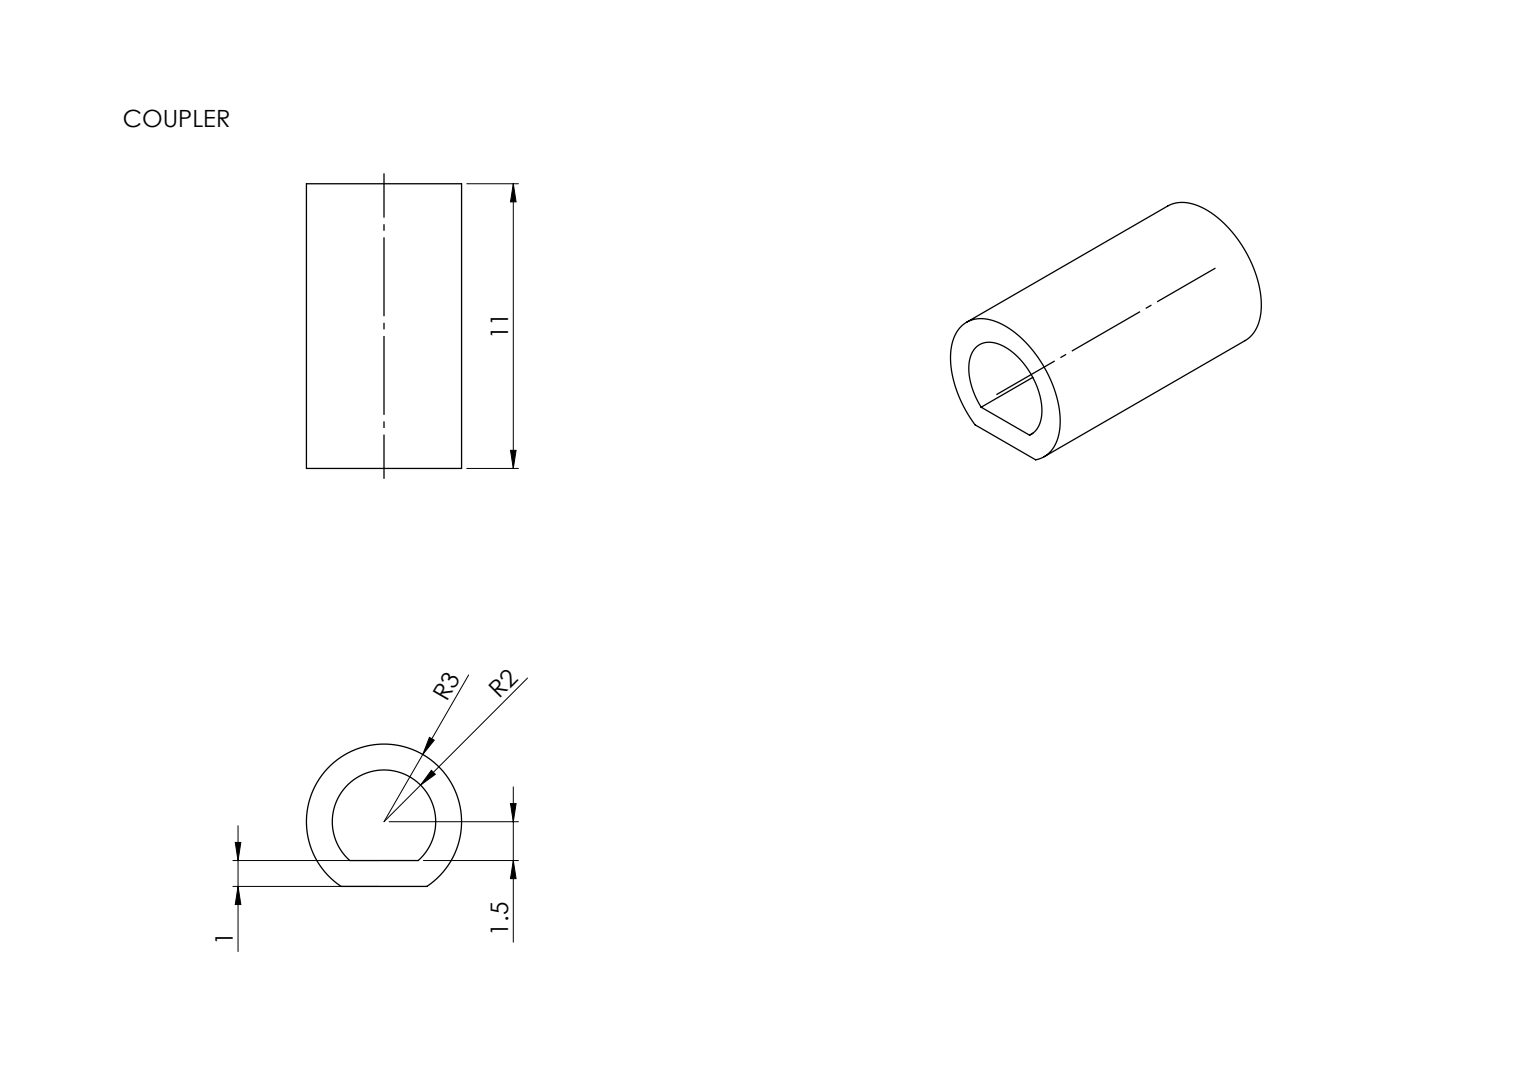
ISO-10303-21;
HEADER;
FILE_DESCRIPTION (('STEP AP214'),
    '1' );
FILE_NAME ('coupler.step',
    '2026-10-02T09:26:43',
    ( '' ),
    ( '' ),
    'SwSTEP 2.0',
    'SolidWorks 2026',
    '' );
FILE_SCHEMA (( 'AUTOMOTIVE_DESIGN' ));
ENDSEC;

DATA;
#121=CARTESIAN_POINT ( 'NONE',  ( -3.000000000000000000, 3.673940397442059868E-16, -5.000000000000004441 ) ) ;
#140=FACE_OUTER_BOUND ( 'NONE', #29426, .T. ) ;
#510=CARTESIAN_POINT ( 'NONE',  ( 0.000000000000000000, 0.000000000000000000, 6.000000000000005329 ) ) ;
#797=DIRECTION ( 'NONE',  ( 0.000000000000000000, -1.000000000000000000, 0.000000000000000000 ) ) ;
#830=EDGE_CURVE ( 'NONE', #63242, #121356, #72655, .T. ) ;
#3162=DIRECTION ( 'NONE',  ( 1.000000000000000000, 0.000000000000000000, 0.000000000000000000 ) ) ;
#3336=EDGE_CURVE ( 'NONE', #106026, #55502, #20118, .T. ) ;
#3524=CARTESIAN_POINT ( 'NONE',  ( -3.000000000000000000, 3.673940397442059868E-16, 6.000000000000005329 ) ) ;
#3829=VECTOR ( 'NONE', #31652, 1000.000000000000000 ) ;
#3916=SHAPE_REPRESENTATION_RELATIONSHIP ( 'NONE' , 'NONE' ,  #71195, #50879 ) ;
#4519=PRODUCT_DEFINITION_FORMATION_WITH_SPECIFIED_SOURCE ( 'ANY', '', #111975, .NOT_KNOWN. ) ;
#5236=PRODUCT_DEFINITION ( 'UNKNOWN', '', #4519, #49332 ) ;
#5531=AXIS2_PLACEMENT_3D ( 'NONE', #87883, #67606, #9346 ) ;
#5667=AXIS2_PLACEMENT_3D ( 'NONE', #39891, #58867, #98137 ) ;
#5700=CARTESIAN_POINT ( 'NONE',  ( -1.322875655532295136, -1.500000000000000222, 6.000000000000005329 ) ) ;
#5791=EDGE_LOOP ( 'NONE', ( #54468, #103310, #17198, #105823 ) ) ;
#6026=AXIS2_PLACEMENT_3D ( 'NONE', #62055, #31948, #71212 ) ;
#6057=FILL_AREA_STYLE_COLOUR ( '', #69146 ) ;
#6824=DIRECTION ( 'NONE',  ( 0.000000000000000000, 0.000000000000000000, 1.000000000000000000 ) ) ;
#6973=EDGE_CURVE ( 'NONE', #15557, #33416, #50411, .T. ) ;
#7096=EDGE_CURVE ( 'NONE', #113294, #58747, #13842, .T. ) ;
#7288=ORIENTED_EDGE ( 'NONE', *, *, #129076, .T. ) ;
#7517=CIRCLE ( 'NONE', #99487, 2.000000000000000000 ) ;
#8386=EDGE_LOOP ( 'NONE', ( #21515, #31620, #80877, #68622 ) ) ;
#8391=ADVANCED_FACE ( 'NONE', ( #66505 ), #113691, .T. ) ;
#8628=PRESENTATION_STYLE_ASSIGNMENT (( #46012 ) ) ;
#9105=VERTEX_POINT ( 'NONE', #120623 ) ;
#9346=DIRECTION ( 'NONE',  ( 1.000000000000000000, 0.000000000000000000, 0.000000000000000000 ) ) ;
#10644=CARTESIAN_POINT ( 'NONE',  ( 0.000000000000000000, 0.000000000000000000, 0.000000000000000000 ) ) ;
#10879=ORIENTED_EDGE ( 'NONE', *, *, #26098, .F. ) ;
#11137=DIRECTION ( 'NONE',  ( 0.000000000000000000, 0.000000000000000000, -1.000000000000000000 ) ) ;
#11803=VECTOR ( 'NONE', #66278, 1000.000000000000000 ) ;
#12273=CARTESIAN_POINT ( 'NONE',  ( 0.000000000000000000, 0.000000000000000000, 6.000000000000005329 ) ) ;
#12515=CARTESIAN_POINT ( 'NONE',  ( 0.000000000000000000, 0.000000000000000000, 6.000000000000005329 ) ) ;
#12752=VERTEX_POINT ( 'NONE', #40215 ) ;
#13727=PRESENTATION_STYLE_ASSIGNMENT (( #105348 ) ) ;
#13796=EDGE_CURVE ( 'NONE', #113294, #14153, #20257, .T. ) ;
#13842=CIRCLE ( 'NONE', #95430, 3.000000000000000000 ) ;
#14153=VERTEX_POINT ( 'NONE', #3524 ) ;
#14367=FILL_AREA_STYLE_COLOUR ( '', #49923 ) ;
#15427=DIRECTION ( 'NONE',  ( 0.000000000000000000, 0.000000000000000000, 1.000000000000000000 ) ) ;
#15480=ORIENTED_EDGE ( 'NONE', *, *, #26098, .T. ) ;
#15494=CARTESIAN_POINT ( 'NONE',  ( 0.000000000000000000, 0.000000000000000000, -5.000000000000004441 ) ) ;
#15557=VERTEX_POINT ( 'NONE', #69207 ) ;
#15625=EDGE_LOOP ( 'NONE', ( #57211, #65939, #124671, #93586 ) ) ;
#15810=VECTOR ( 'NONE', #20956, 1000.000000000000000 ) ;
#16030=ADVANCED_FACE ( 'NONE', ( #40541 ), #18290, .F. ) ;
#16169=AXIS2_PLACEMENT_3D ( 'NONE', #75260, #26171, #96181 ) ;
#16469=ORIENTED_EDGE ( 'NONE', *, *, #30069, .F. ) ;
#16559=FACE_BOUND ( 'NONE', #42887, .T. ) ;
#16568=EDGE_CURVE ( 'NONE', #33416, #14153, #125380, .T. ) ;
#16696=EDGE_LOOP ( 'NONE', ( #90752, #119802, #97487, #87277 ) ) ;
#16932=VERTEX_POINT ( 'NONE', #51031 ) ;
#17198=ORIENTED_EDGE ( 'NONE', *, *, #76465, .F. ) ;
#18290=CYLINDRICAL_SURFACE ( 'NONE', #5667, 2.000000000000000000 ) ;
#18737=ORIENTED_EDGE ( 'NONE', *, *, #42194, .F. ) ;
#18894=ORIENTED_EDGE ( 'NONE', *, *, #67726, .F. ) ;
#19635=FACE_OUTER_BOUND ( 'NONE', #8386, .T. ) ;
#20118=CIRCLE ( 'NONE', #16169, 2.000000000000000000 ) ;
#20257=LINE ( 'NONE', #113632, #62540 ) ;
#20956=DIRECTION ( 'NONE',  ( 0.000000000000000000, 0.000000000000000000, 1.000000000000000000 ) ) ;
#21257=EDGE_CURVE ( 'NONE', #14153, #63242, #113529, .T. ) ;
#21274=VERTEX_POINT ( 'NONE', #79105 ) ;
#21515=ORIENTED_EDGE ( 'NONE', *, *, #13796, .F. ) ;
#21809=CARTESIAN_POINT ( 'NONE',  ( 0.000000000000000000, 0.000000000000000000, 6.000000000000005329 ) ) ;
#22053=AXIS2_PLACEMENT_3D ( 'NONE', #65765, #6824, #24563 ) ;
#22460=DIRECTION ( 'NONE',  ( 0.000000000000000000, 0.000000000000000000, 1.000000000000000000 ) ) ;
#23295=LINE ( 'NONE', #110392, #33797 ) ;
#23792=CARTESIAN_POINT ( 'NONE',  ( 1.322875655532295136, -1.500000000000000222, -5.000000000000004441 ) ) ;
#24563=DIRECTION ( 'NONE',  ( 1.000000000000000000, 0.000000000000000000, 0.000000000000000000 ) ) ;
#24625=APPLICATION_CONTEXT ( 'automotive_design' ) ;
#25196=VECTOR ( 'NONE', #34094, 1000.000000000000000 ) ;
#25601=CIRCLE ( 'NONE', #63187, 2.000000000000000000 ) ;
#26098=EDGE_CURVE ( 'NONE', #15557, #113294, #55419, .T. ) ;
#26171=DIRECTION ( 'NONE',  ( 0.000000000000000000, 0.000000000000000000, 1.000000000000000000 ) ) ;
#26869=DIRECTION ( 'NONE',  ( 1.000000000000000000, 0.000000000000000000, 0.000000000000000000 ) ) ;
#26920=ORIENTED_EDGE ( 'NONE', *, *, #77354, .F. ) ;
#27012=SURFACE_SIDE_STYLE ('',( #58415 ) ) ;
#28342=DIRECTION ( 'NONE',  ( 0.000000000000000000, 0.000000000000000000, -1.000000000000000000 ) ) ;
#28589=EDGE_CURVE ( 'NONE', #16932, #21274, #25601, .T. ) ;
#28709=DIRECTION ( 'NONE',  ( 0.000000000000000000, 0.000000000000000000, 1.000000000000000000 ) ) ;
#28826=AXIS2_PLACEMENT_3D ( 'NONE', #15494, #115628, #103896 ) ;
#28851=AXIS2_PLACEMENT_3D ( 'NONE', #35147, #44955, #56039 ) ;
#28949=ORIENTED_EDGE ( 'NONE', *, *, #117304, .F. ) ;
#28951=LINE ( 'NONE', #86559, #11803 ) ;
#29426=EDGE_LOOP ( 'NONE', ( #127737, #47956, #18737, #67731 ) ) ;
#29661=ORIENTED_EDGE ( 'NONE', *, *, #3336, .T. ) ;
#30069=EDGE_CURVE ( 'NONE', #61997, #15557, #65779, .T. ) ;
#31620=ORIENTED_EDGE ( 'NONE', *, *, #7096, .T. ) ;
#31652=DIRECTION ( 'NONE',  ( 1.000000000000000000, 0.000000000000000000, 0.000000000000000000 ) ) ;
#31948=DIRECTION ( 'NONE',  ( 0.000000000000000000, 0.000000000000000000, 1.000000000000000000 ) ) ;
#32102=DIRECTION ( 'NONE',  ( 0.000000000000000000, -1.000000000000000000, 0.000000000000000000 ) ) ;
#33280=DIRECTION ( 'NONE',  ( 0.000000000000000000, 0.000000000000000000, 1.000000000000000000 ) ) ;
#33402=( NAMED_UNIT ( * ) PLANE_ANGLE_UNIT ( ) SI_UNIT ( $, .RADIAN. ) );
#33416=VERTEX_POINT ( 'NONE', #37331 ) ;
#33552=DIRECTION ( 'NONE',  ( 0.000000000000000000, 0.000000000000000000, 1.000000000000000000 ) ) ;
#33797=VECTOR ( 'NONE', #92044, 1000.000000000000000 ) ;
#33972=EDGE_LOOP ( 'NONE', ( #15480, #69240, #68935, #118863 ) ) ;
#34094=DIRECTION ( 'NONE',  ( 0.000000000000000000, 0.000000000000000000, 1.000000000000000000 ) ) ;
#34695=CARTESIAN_POINT ( 'NONE',  ( -1.658312395177699017, -2.500000000000000444, 6.000000000000005329 ) ) ;
#34746=ADVANCED_FACE ( 'NONE', ( #19635 ), #79830, .T. ) ;
#35092=DIRECTION ( 'NONE',  ( 1.000000000000000000, 0.000000000000000000, 0.000000000000000000 ) ) ;
#35147=CARTESIAN_POINT ( 'NONE',  ( 0.000000000000000000, 0.000000000000000000, -5.000000000000004441 ) ) ;
#35414=LINE ( 'NONE', #125072, #105460 ) ;
#37331=CARTESIAN_POINT ( 'NONE',  ( 3.000000000000000000, 0.000000000000000000, 6.000000000000005329 ) ) ;
#37649=PRODUCT_DEFINITION_SHAPE ( 'NONE', 'NONE',  #5236 ) ;
#37995=APPLICATION_CONTEXT ( 'automotive_design' ) ;
#38839=CYLINDRICAL_SURFACE ( 'NONE', #5531, 2.000000000000000000 ) ;
#39891=CARTESIAN_POINT ( 'NONE',  ( 0.000000000000000000, 0.000000000000000000, -5.000000000000004441 ) ) ;
#40215=CARTESIAN_POINT ( 'NONE',  ( 1.322875655532295136, -1.500000000000000222, 6.000000000000005329 ) ) ;
#40409=CARTESIAN_POINT ( 'NONE',  ( -2.000000000000000000, 2.449293598294706414E-16, 6.000000000000005329 ) ) ;
#40541=FACE_OUTER_BOUND ( 'NONE', #15625, .T. ) ;
#40667=ORIENTED_EDGE ( 'NONE', *, *, #122642, .T. ) ;
#41296=AXIS2_PLACEMENT_3D ( 'NONE', #21809, #22460, #51910 ) ;
#42194=EDGE_CURVE ( 'NONE', #58747, #63242, #35414, .T. ) ;
#42640=EDGE_CURVE ( 'NONE', #21274, #106026, #65167, .T. ) ;
#42657=DIRECTION ( 'NONE',  ( 0.000000000000000000, 0.000000000000000000, 1.000000000000000000 ) ) ;
#42887=EDGE_LOOP ( 'NONE', ( #18894, #74442, #28949, #116817 ) ) ;
#43089=ADVANCED_FACE ( 'NONE', ( #65011, #16559 ), #86602, .T. ) ;
#43736=LINE ( 'NONE', #5700, #55418 ) ;
#43866=SURFACE_STYLE_FILL_AREA ( #84413 ) ;
#44955=DIRECTION ( 'NONE',  ( 0.000000000000000000, 0.000000000000000000, 1.000000000000000000 ) ) ;
#44985=CYLINDRICAL_SURFACE ( 'NONE', #28826, 3.000000000000000000 ) ;
#45200=ORIENTED_EDGE ( 'NONE', *, *, #86954, .F. ) ;
#45468=AXIS2_PLACEMENT_3D ( 'NONE', #12273, #60750, #103252 ) ;
#45745=EDGE_LOOP ( 'NONE', ( #40667, #7288, #88586, #87697 ) ) ;
#45875=CARTESIAN_POINT ( 'NONE',  ( 0.000000000000000000, 0.000000000000000000, -5.000000000000004441 ) ) ;
#46012=SURFACE_STYLE_USAGE ( .BOTH. , #27012 ) ;
#46496=CYLINDRICAL_SURFACE ( 'NONE', #128338, 2.000000000000000000 ) ;
#46647=( NAMED_UNIT ( * ) PLANE_ANGLE_UNIT ( ) SI_UNIT ( $, .RADIAN. ) );
#46771=VECTOR ( 'NONE', #35092, 1000.000000000000000 ) ;
#47956=ORIENTED_EDGE ( 'NONE', *, *, #830, .F. ) ;
#48256=CARTESIAN_POINT ( 'NONE',  ( -1.322875655532295136, -1.500000000000000222, -5.000000000000004441 ) ) ;
#48698=ADVANCED_FACE ( 'NONE', ( #140 ), #69535, .T. ) ;
#48839=AXIS2_PLACEMENT_3D ( 'NONE', #102687, #62788, #73241 ) ;
#49332=PRODUCT_DEFINITION_CONTEXT ( 'detailed design', #24625, 'design' ) ;
#49923=COLOUR_RGB ( '', 0.31764706, 0.68627451, 0.89019608) ;
#50411=LINE ( 'NONE', #110621, #15810 ) ;
#50879=ADVANCED_BREP_SHAPE_REPRESENTATION ( '', ( #102059, #108296 ), #66615 ) ;
#51031=CARTESIAN_POINT ( 'NONE',  ( 2.000000000000000000, 0.000000000000000000, -5.000000000000004441 ) ) ;
#51805=LINE ( 'NONE', #113280, #25196 ) ;
#51910=DIRECTION ( 'NONE',  ( 1.000000000000000000, 0.000000000000000000, 0.000000000000000000 ) ) ;
#54468=ORIENTED_EDGE ( 'NONE', *, *, #77354, .T. ) ;
#54686=CARTESIAN_POINT ( 'NONE',  ( -1.322875655532295136, -2.500000000000000444, -5.000000000000004441 ) ) ;
#55093=DIRECTION ( 'NONE',  ( 1.000000000000000000, 0.000000000000000000, 0.000000000000000000 ) ) ;
#55418=VECTOR ( 'NONE', #73174, 1000.000000000000000 ) ;
#55419=CIRCLE ( 'NONE', #93078, 3.000000000000000000 ) ;
#55502=VERTEX_POINT ( 'NONE', #76988 ) ;
#55575=DIRECTION ( 'NONE',  ( 1.000000000000000000, 0.000000000000000000, 0.000000000000000000 ) ) ;
#55759=ORIENTED_EDGE ( 'NONE', *, *, #7096, .F. ) ;
#56004=CARTESIAN_POINT ( 'NONE',  ( -2.000000000000000000, 2.449293598294706414E-16, -5.000000000000004441 ) ) ;
#56039=DIRECTION ( 'NONE',  ( 1.000000000000000000, 0.000000000000000000, 0.000000000000000000 ) ) ;
#56171=ADVANCED_FACE ( 'NONE', ( #61557 ), #72662, .F. ) ;
#56497=EDGE_CURVE ( 'NONE', #121356, #33416, #57977, .T. ) ;
#56639=ADVANCED_FACE ( 'NONE', ( #75078 ), #44985, .T. ) ;
#56862=DIRECTION ( 'NONE',  ( 1.000000000000000000, 0.000000000000000000, 0.000000000000000000 ) ) ;
#56949=FACE_OUTER_BOUND ( 'NONE', #128515, .T. ) ;
#57211=ORIENTED_EDGE ( 'NONE', *, *, #112117, .F. ) ;
#57977=CIRCLE ( 'NONE', #45468, 3.000000000000000000 ) ;
#58415=SURFACE_STYLE_FILL_AREA ( #127777 ) ;
#58747=VERTEX_POINT ( 'NONE', #58949 ) ;
#58867=DIRECTION ( 'NONE',  ( 0.000000000000000000, 0.000000000000000000, 1.000000000000000000 ) ) ;
#58949=CARTESIAN_POINT ( 'NONE',  ( -1.658312395177699017, -2.500000000000000444, -5.000000000000004441 ) ) ;
#58992=EDGE_CURVE ( 'NONE', #58747, #61997, #83540, .T. ) ;
#59479=DIRECTION ( 'NONE',  ( 1.000000000000000000, 0.000000000000000000, 0.000000000000000000 ) ) ;
#60394=CARTESIAN_POINT ( 'NONE',  ( -1.322875655532295136, -2.500000000000000444, -5.000000000000004441 ) ) ;
#60750=DIRECTION ( 'NONE',  ( 0.000000000000000000, 0.000000000000000000, 1.000000000000000000 ) ) ;
#60816=ADVANCED_FACE ( 'NONE', ( #128505 ), #38839, .F. ) ;
#61198=DIRECTION ( 'NONE',  ( 0.000000000000000000, 0.000000000000000000, 1.000000000000000000 ) ) ;
#61557=FACE_OUTER_BOUND ( 'NONE', #5791, .T. ) ;
#61997=VERTEX_POINT ( 'NONE', #122067 ) ;
#62055=CARTESIAN_POINT ( 'NONE',  ( 0.000000000000000000, 0.000000000000000000, -5.000000000000004441 ) ) ;
#62540=VECTOR ( 'NONE', #99475, 1000.000000000000000 ) ;
#62788=DIRECTION ( 'NONE',  ( 0.000000000000000000, 0.000000000000000000, 1.000000000000000000 ) ) ;
#63187=AXIS2_PLACEMENT_3D ( 'NONE', #126277, #124346, #56862 ) ;
#63242=VERTEX_POINT ( 'NONE', #34695 ) ;
#63328=FACE_BOUND ( 'NONE', #45745, .T. ) ;
#63794=VECTOR ( 'NONE', #15427, 1000.000000000000000 ) ;
#63815=CIRCLE ( 'NONE', #22053, 2.000000000000000000 ) ;
#64736=VECTOR ( 'NONE', #33552, 1000.000000000000000 ) ;
#64852=DIRECTION ( 'NONE',  ( 0.000000000000000000, 0.000000000000000000, 1.000000000000000000 ) ) ;
#64894=CARTESIAN_POINT ( 'NONE',  ( 0.000000000000000000, 0.000000000000000000, -5.000000000000004441 ) ) ;
#65011=FACE_OUTER_BOUND ( 'NONE', #110996, .T. ) ;
#65167=LINE ( 'NONE', #56004, #63794 ) ;
#65765=CARTESIAN_POINT ( 'NONE',  ( 0.000000000000000000, 0.000000000000000000, 6.000000000000005329 ) ) ;
#65779=CIRCLE ( 'NONE', #122239, 3.000000000000000000 ) ;
#65939=ORIENTED_EDGE ( 'NONE', *, *, #129076, .F. ) ;
#66139=DIRECTION ( 'NONE',  ( 0.000000000000000000, 0.000000000000000000, 1.000000000000000000 ) ) ;
#66278=DIRECTION ( 'NONE',  ( 0.000000000000000000, 0.000000000000000000, 1.000000000000000000 ) ) ;
#66281=( LENGTH_UNIT ( ) NAMED_UNIT ( * ) SI_UNIT ( .MILLI., .METRE. ) );
#66505=FACE_OUTER_BOUND ( 'NONE', #33972, .T. ) ;
#66615=( GEOMETRIC_REPRESENTATION_CONTEXT ( 3 ) GLOBAL_UNCERTAINTY_ASSIGNED_CONTEXT ( ( #114463 ) ) GLOBAL_UNIT_ASSIGNED_CONTEXT ( ( #80562, #33402, #74597 ) ) REPRESENTATION_CONTEXT ( 'NONE', 'WORKASPACE' ) );
#66692=ORIENTED_EDGE ( 'NONE', *, *, #123717, .F. ) ;
#66912=( NAMED_UNIT ( * ) SI_UNIT ( $, .STERADIAN. ) SOLID_ANGLE_UNIT ( ) );
#67606=DIRECTION ( 'NONE',  ( 0.000000000000000000, 0.000000000000000000, 1.000000000000000000 ) ) ;
#67726=EDGE_CURVE ( 'NONE', #55502, #12752, #43736, .T. ) ;
#67731=ORIENTED_EDGE ( 'NONE', *, *, #58992, .T. ) ;
#67986=SHAPE_DEFINITION_REPRESENTATION ( #37649, #71195 ) ;
#68622=ORIENTED_EDGE ( 'NONE', *, *, #21257, .F. ) ;
#68935=ORIENTED_EDGE ( 'NONE', *, *, #16568, .F. ) ;
#69146=COLOUR_RGB ( '', 0.31764706, 0.68627451, 0.89019608) ;
#69207=CARTESIAN_POINT ( 'NONE',  ( 3.000000000000000000, 0.000000000000000000, -5.000000000000004441 ) ) ;
#69240=ORIENTED_EDGE ( 'NONE', *, *, #13796, .T. ) ;
#69535=PLANE ( 'NONE',  #115343 ) ;
#70718=CARTESIAN_POINT ( 'NONE',  ( -1.322875655532295136, -1.500000000000000222, -5.000000000000004441 ) ) ;
#71195=SHAPE_REPRESENTATION ( 'coupler', ( #108296 ), #66615 ) ;
#71212=DIRECTION ( 'NONE',  ( 1.000000000000000000, 0.000000000000000000, 0.000000000000000000 ) ) ;
#72655=LINE ( 'NONE', #104041, #73376 ) ;
#72662=PLANE ( 'NONE',  #105998 ) ;
#73174=DIRECTION ( 'NONE',  ( 1.000000000000000000, 0.000000000000000000, 0.000000000000000000 ) ) ;
#73241=DIRECTION ( 'NONE',  ( 1.000000000000000000, 0.000000000000000000, 0.000000000000000000 ) ) ;
#73376=VECTOR ( 'NONE', #104662, 1000.000000000000000 ) ;
#73996=ORIENTED_EDGE ( 'NONE', *, *, #42640, .T. ) ;
#74442=ORIENTED_EDGE ( 'NONE', *, *, #3336, .F. ) ;
#74473=CARTESIAN_POINT ( 'NONE',  ( 0.000000000000000000, 0.000000000000000000, -5.000000000000004441 ) ) ;
#74597=( NAMED_UNIT ( * ) SI_UNIT ( $, .STERADIAN. ) SOLID_ANGLE_UNIT ( ) );
#75078=FACE_OUTER_BOUND ( 'NONE', #116314, .T. ) ;
#75260=CARTESIAN_POINT ( 'NONE',  ( 0.000000000000000000, 0.000000000000000000, 6.000000000000005329 ) ) ;
#75414=( GEOMETRIC_REPRESENTATION_CONTEXT ( 3 ) GLOBAL_UNCERTAINTY_ASSIGNED_CONTEXT ( ( #75436 ) ) GLOBAL_UNIT_ASSIGNED_CONTEXT ( ( #66281, #46647, #66912 ) ) REPRESENTATION_CONTEXT ( 'NONE', 'WORKASPACE' ) );
#75436=UNCERTAINTY_MEASURE_WITH_UNIT (LENGTH_MEASURE( 1.000000000000000082E-05 ), #66281, 'distance_accuracy_value', 'NONE');
#75488=DIRECTION ( 'NONE',  ( 1.000000000000000000, 0.000000000000000000, 0.000000000000000000 ) ) ;
#75878=( NAMED_UNIT ( * ) SI_UNIT ( $, .STERADIAN. ) SOLID_ANGLE_UNIT ( ) );
#76465=EDGE_CURVE ( 'NONE', #118978, #12752, #51805, .T. ) ;
#76537=PRODUCT_CONTEXT ( 'NONE', #37995, 'mechanical' ) ;
#76988=CARTESIAN_POINT ( 'NONE',  ( -1.322875655532295136, -1.500000000000000222, 6.000000000000005329 ) ) ;
#77248=VERTEX_POINT ( 'NONE', #48256 ) ;
#77354=EDGE_CURVE ( 'NONE', #77248, #55502, #23295, .T. ) ;
#78913=ORIENTED_EDGE ( 'NONE', *, *, #30069, .T. ) ;
#79018=ORIENTED_EDGE ( 'NONE', *, *, #21257, .T. ) ;
#79105=CARTESIAN_POINT ( 'NONE',  ( -2.000000000000000000, 2.449293598294706414E-16, -5.000000000000004441 ) ) ;
#79830=CYLINDRICAL_SURFACE ( 'NONE', #48839, 3.000000000000000000 ) ;
#80562=( LENGTH_UNIT ( ) NAMED_UNIT ( * ) SI_UNIT ( .MILLI., .METRE. ) );
#80718=DIRECTION ( 'NONE',  ( 1.000000000000000000, 0.000000000000000000, 0.000000000000000000 ) ) ;
#80877=ORIENTED_EDGE ( 'NONE', *, *, #42194, .T. ) ;
#81409=LINE ( 'NONE', #121315, #3829 ) ;
#83540=LINE ( 'NONE', #54686, #46771 ) ;
#83597=CIRCLE ( 'NONE', #123295, 2.000000000000000000 ) ;
#84413=FILL_AREA_STYLE ('',( #14367 ) ) ;
#84555=EDGE_CURVE ( 'NONE', #12752, #9105, #129131, .T. ) ;
#85662=AXIS2_PLACEMENT_3D ( 'NONE', #12515, #42657, #104133 ) ;
#85695=SURFACE_SIDE_STYLE ('',( #43866 ) ) ;
#85869=STYLED_ITEM ( 'NONE', ( #8628 ), #102059 ) ;
#86559=CARTESIAN_POINT ( 'NONE',  ( 2.000000000000000000, 0.000000000000000000, -5.000000000000004441 ) ) ;
#86602=PLANE ( 'NONE',  #86855 ) ;
#86855=AXIS2_PLACEMENT_3D ( 'NONE', #97076, #116066, #75488 ) ;
#86954=EDGE_CURVE ( 'NONE', #21274, #77248, #83597, .T. ) ;
#87277=ORIENTED_EDGE ( 'NONE', *, *, #117304, .T. ) ;
#87697=ORIENTED_EDGE ( 'NONE', *, *, #86954, .T. ) ;
#87883=CARTESIAN_POINT ( 'NONE',  ( 0.000000000000000000, 0.000000000000000000, -5.000000000000004441 ) ) ;
#88167=ORIENTED_EDGE ( 'NONE', *, *, #16568, .T. ) ;
#88586=ORIENTED_EDGE ( 'NONE', *, *, #28589, .T. ) ;
#90516=DIRECTION ( 'NONE',  ( 0.000000000000000000, 0.000000000000000000, 1.000000000000000000 ) ) ;
#90752=ORIENTED_EDGE ( 'NONE', *, *, #42640, .F. ) ;
#91305=EDGE_LOOP ( 'NONE', ( #16469, #127192, #55759, #10879 ) ) ;
#91668=STYLED_ITEM ( 'NONE', ( #13727 ), #50879 ) ;
#91891=ORIENTED_EDGE ( 'NONE', *, *, #56497, .F. ) ;
#92044=DIRECTION ( 'NONE',  ( 0.000000000000000000, 0.000000000000000000, 1.000000000000000000 ) ) ;
#92832=DIRECTION ( 'NONE',  ( 1.000000000000000000, 0.000000000000000000, 0.000000000000000000 ) ) ;
#93078=AXIS2_PLACEMENT_3D ( 'NONE', #96748, #61198, #126880 ) ;
#93436=FACE_OUTER_BOUND ( 'NONE', #91305, .T. ) ;
#93586=ORIENTED_EDGE ( 'NONE', *, *, #84555, .T. ) ;
#94854=CARTESIAN_POINT ( 'NONE',  ( 0.000000000000000000, 0.000000000000000000, -5.000000000000004441 ) ) ;
#95031=ADVANCED_FACE ( 'NONE', ( #56949 ), #46496, .F. ) ;
#95430=AXIS2_PLACEMENT_3D ( 'NONE', #94854, #112570, #55575 ) ;
#95878=MECHANICAL_DESIGN_GEOMETRIC_PRESENTATION_REPRESENTATION('',(#91668),#123068);
#96181=DIRECTION ( 'NONE',  ( 1.000000000000000000, 0.000000000000000000, 0.000000000000000000 ) ) ;
#96336=MECHANICAL_DESIGN_GEOMETRIC_PRESENTATION_REPRESENTATION('',(#85869),#75414);
#96748=CARTESIAN_POINT ( 'NONE',  ( 0.000000000000000000, 0.000000000000000000, -5.000000000000004441 ) ) ;
#97076=CARTESIAN_POINT ( 'NONE',  ( 0.000000000000000000, 0.000000000000000000, 6.000000000000005329 ) ) ;
#97487=ORIENTED_EDGE ( 'NONE', *, *, #112117, .T. ) ;
#98137=DIRECTION ( 'NONE',  ( 1.000000000000000000, 0.000000000000000000, 0.000000000000000000 ) ) ;
#99475=DIRECTION ( 'NONE',  ( 0.000000000000000000, 0.000000000000000000, 1.000000000000000000 ) ) ;
#99487=AXIS2_PLACEMENT_3D ( 'NONE', #64894, #104811, #55093 ) ;
#99554=ORIENTED_EDGE ( 'NONE', *, *, #830, .T. ) ;
#101008=AXIS2_PLACEMENT_3D ( 'NONE', #510, #28709, #59479 ) ;
#102059=MANIFOLD_SOLID_BREP ( 'Extrude-Thin1', #112600 ) ;
#102687=CARTESIAN_POINT ( 'NONE',  ( 0.000000000000000000, 0.000000000000000000, -5.000000000000004441 ) ) ;
#103252=DIRECTION ( 'NONE',  ( 1.000000000000000000, 0.000000000000000000, 0.000000000000000000 ) ) ;
#103292=DIRECTION ( 'NONE',  ( 0.000000000000000000, 0.000000000000000000, 1.000000000000000000 ) ) ;
#103310=ORIENTED_EDGE ( 'NONE', *, *, #67726, .T. ) ;
#103418=( LENGTH_UNIT ( ) NAMED_UNIT ( * ) SI_UNIT ( .MILLI., .METRE. ) );
#103896=DIRECTION ( 'NONE',  ( 1.000000000000000000, 0.000000000000000000, 0.000000000000000000 ) ) ;
#103931=CARTESIAN_POINT ( 'NONE',  ( 0.000000000000000000, 0.000000000000000000, -5.000000000000004441 ) ) ;
#104041=CARTESIAN_POINT ( 'NONE',  ( -1.322875655532295136, -2.500000000000000444, 6.000000000000005329 ) ) ;
#104133=DIRECTION ( 'NONE',  ( 1.000000000000000000, 0.000000000000000000, 0.000000000000000000 ) ) ;
#104662=DIRECTION ( 'NONE',  ( 1.000000000000000000, 0.000000000000000000, 0.000000000000000000 ) ) ;
#104811=DIRECTION ( 'NONE',  ( 0.000000000000000000, 0.000000000000000000, 1.000000000000000000 ) ) ;
#105348=SURFACE_STYLE_USAGE ( .BOTH. , #85695 ) ;
#105460=VECTOR ( 'NONE', #64852, 1000.000000000000000 ) ;
#105543=UNCERTAINTY_MEASURE_WITH_UNIT (LENGTH_MEASURE( 1.000000000000000082E-05 ), #103418, 'distance_accuracy_value', 'NONE');
#105823=ORIENTED_EDGE ( 'NONE', *, *, #122642, .F. ) ;
#105998=AXIS2_PLACEMENT_3D ( 'NONE', #70718, #32102, #11137 ) ;
#106026=VERTEX_POINT ( 'NONE', #40409 ) ;
#108296=AXIS2_PLACEMENT_3D ( 'NONE', #10644, #90516, #80718 ) ;
#110392=CARTESIAN_POINT ( 'NONE',  ( -1.322875655532295136, -1.500000000000000222, -5.000000000000004441 ) ) ;
#110621=CARTESIAN_POINT ( 'NONE',  ( 3.000000000000000000, 0.000000000000000000, -5.000000000000004441 ) ) ;
#110996=EDGE_LOOP ( 'NONE', ( #126667, #88167, #79018, #99554 ) ) ;
#111975=PRODUCT ( 'coupler', 'coupler', '', ( #76537 ) ) ;
#112105=CARTESIAN_POINT ( 'NONE',  ( 1.658312395177699017, -2.500000000000000444, -5.000000000000004441 ) ) ;
#112117=EDGE_CURVE ( 'NONE', #16932, #9105, #28951, .T. ) ;
#112570=DIRECTION ( 'NONE',  ( 0.000000000000000000, 0.000000000000000000, 1.000000000000000000 ) ) ;
#112600=CLOSED_SHELL ( 'NONE', ( #95031, #60816, #8391, #56639, #34746, #48698, #120796, #16030, #56171, #43089 ) ) ;
#113280=CARTESIAN_POINT ( 'NONE',  ( 1.322875655532295136, -1.500000000000000222, -5.000000000000004441 ) ) ;
#113294=VERTEX_POINT ( 'NONE', #121 ) ;
#113529=CIRCLE ( 'NONE', #101008, 3.000000000000000000 ) ;
#113632=CARTESIAN_POINT ( 'NONE',  ( -3.000000000000000000, 3.673940397442059868E-16, -5.000000000000004441 ) ) ;
#113691=CYLINDRICAL_SURFACE ( 'NONE', #28851, 3.000000000000000000 ) ;
#114463=UNCERTAINTY_MEASURE_WITH_UNIT (LENGTH_MEASURE( 1.000000000000000082E-05 ), #80562, 'distance_accuracy_value', 'NONE');
#114508=( NAMED_UNIT ( * ) PLANE_ANGLE_UNIT ( ) SI_UNIT ( $, .RADIAN. ) );
#115343=AXIS2_PLACEMENT_3D ( 'NONE', #60394, #797, #28342 ) ;
#115628=DIRECTION ( 'NONE',  ( 0.000000000000000000, 0.000000000000000000, 1.000000000000000000 ) ) ;
#116066=DIRECTION ( 'NONE',  ( 0.000000000000000000, 0.000000000000000000, 1.000000000000000000 ) ) ;
#116314=EDGE_LOOP ( 'NONE', ( #78913, #128859, #91891, #66692 ) ) ;
#116817=ORIENTED_EDGE ( 'NONE', *, *, #84555, .F. ) ;
#117304=EDGE_CURVE ( 'NONE', #9105, #106026, #63815, .T. ) ;
#118863=ORIENTED_EDGE ( 'NONE', *, *, #6973, .F. ) ;
#118978=VERTEX_POINT ( 'NONE', #23792 ) ;
#119802=ORIENTED_EDGE ( 'NONE', *, *, #28589, .F. ) ;
#120623=CARTESIAN_POINT ( 'NONE',  ( 2.000000000000000000, 0.000000000000000000, 6.000000000000005329 ) ) ;
#120796=ADVANCED_FACE ( 'NONE', ( #63328, #93436 ), #121591, .F. ) ;
#121315=CARTESIAN_POINT ( 'NONE',  ( -1.322875655532295136, -1.500000000000000222, -5.000000000000004441 ) ) ;
#121356=VERTEX_POINT ( 'NONE', #123377 ) ;
#121591=PLANE ( 'NONE',  #6026 ) ;
#122067=CARTESIAN_POINT ( 'NONE',  ( 1.658312395177699017, -2.500000000000000444, -5.000000000000004441 ) ) ;
#122239=AXIS2_PLACEMENT_3D ( 'NONE', #103931, #103292, #92832 ) ;
#122642=EDGE_CURVE ( 'NONE', #77248, #118978, #81409, .T. ) ;
#123068=( GEOMETRIC_REPRESENTATION_CONTEXT ( 3 ) GLOBAL_UNCERTAINTY_ASSIGNED_CONTEXT ( ( #105543 ) ) GLOBAL_UNIT_ASSIGNED_CONTEXT ( ( #103418, #114508, #75878 ) ) REPRESENTATION_CONTEXT ( 'NONE', 'WORKASPACE' ) );
#123214=LINE ( 'NONE', #112105, #64736 ) ;
#123295=AXIS2_PLACEMENT_3D ( 'NONE', #74473, #33280, #3162 ) ;
#123377=CARTESIAN_POINT ( 'NONE',  ( 1.658312395177699017, -2.500000000000000444, 6.000000000000005329 ) ) ;
#123717=EDGE_CURVE ( 'NONE', #61997, #121356, #123214, .T. ) ;
#124346=DIRECTION ( 'NONE',  ( 0.000000000000000000, 0.000000000000000000, 1.000000000000000000 ) ) ;
#124671=ORIENTED_EDGE ( 'NONE', *, *, #76465, .T. ) ;
#125072=CARTESIAN_POINT ( 'NONE',  ( -1.658312395177699017, -2.500000000000000444, -5.000000000000004441 ) ) ;
#125380=CIRCLE ( 'NONE', #85662, 3.000000000000000000 ) ;
#126277=CARTESIAN_POINT ( 'NONE',  ( 0.000000000000000000, 0.000000000000000000, -5.000000000000004441 ) ) ;
#126667=ORIENTED_EDGE ( 'NONE', *, *, #56497, .T. ) ;
#126880=DIRECTION ( 'NONE',  ( 1.000000000000000000, 0.000000000000000000, 0.000000000000000000 ) ) ;
#127192=ORIENTED_EDGE ( 'NONE', *, *, #58992, .F. ) ;
#127737=ORIENTED_EDGE ( 'NONE', *, *, #123717, .T. ) ;
#127777=FILL_AREA_STYLE ('',( #6057 ) ) ;
#128338=AXIS2_PLACEMENT_3D ( 'NONE', #45875, #66139, #26869 ) ;
#128505=FACE_OUTER_BOUND ( 'NONE', #16696, .T. ) ;
#128515=EDGE_LOOP ( 'NONE', ( #45200, #73996, #29661, #26920 ) ) ;
#128859=ORIENTED_EDGE ( 'NONE', *, *, #6973, .T. ) ;
#129076=EDGE_CURVE ( 'NONE', #118978, #16932, #7517, .T. ) ;
#129131=CIRCLE ( 'NONE', #41296, 2.000000000000000000 ) ;
ENDSEC;
END-ISO-10303-21;
